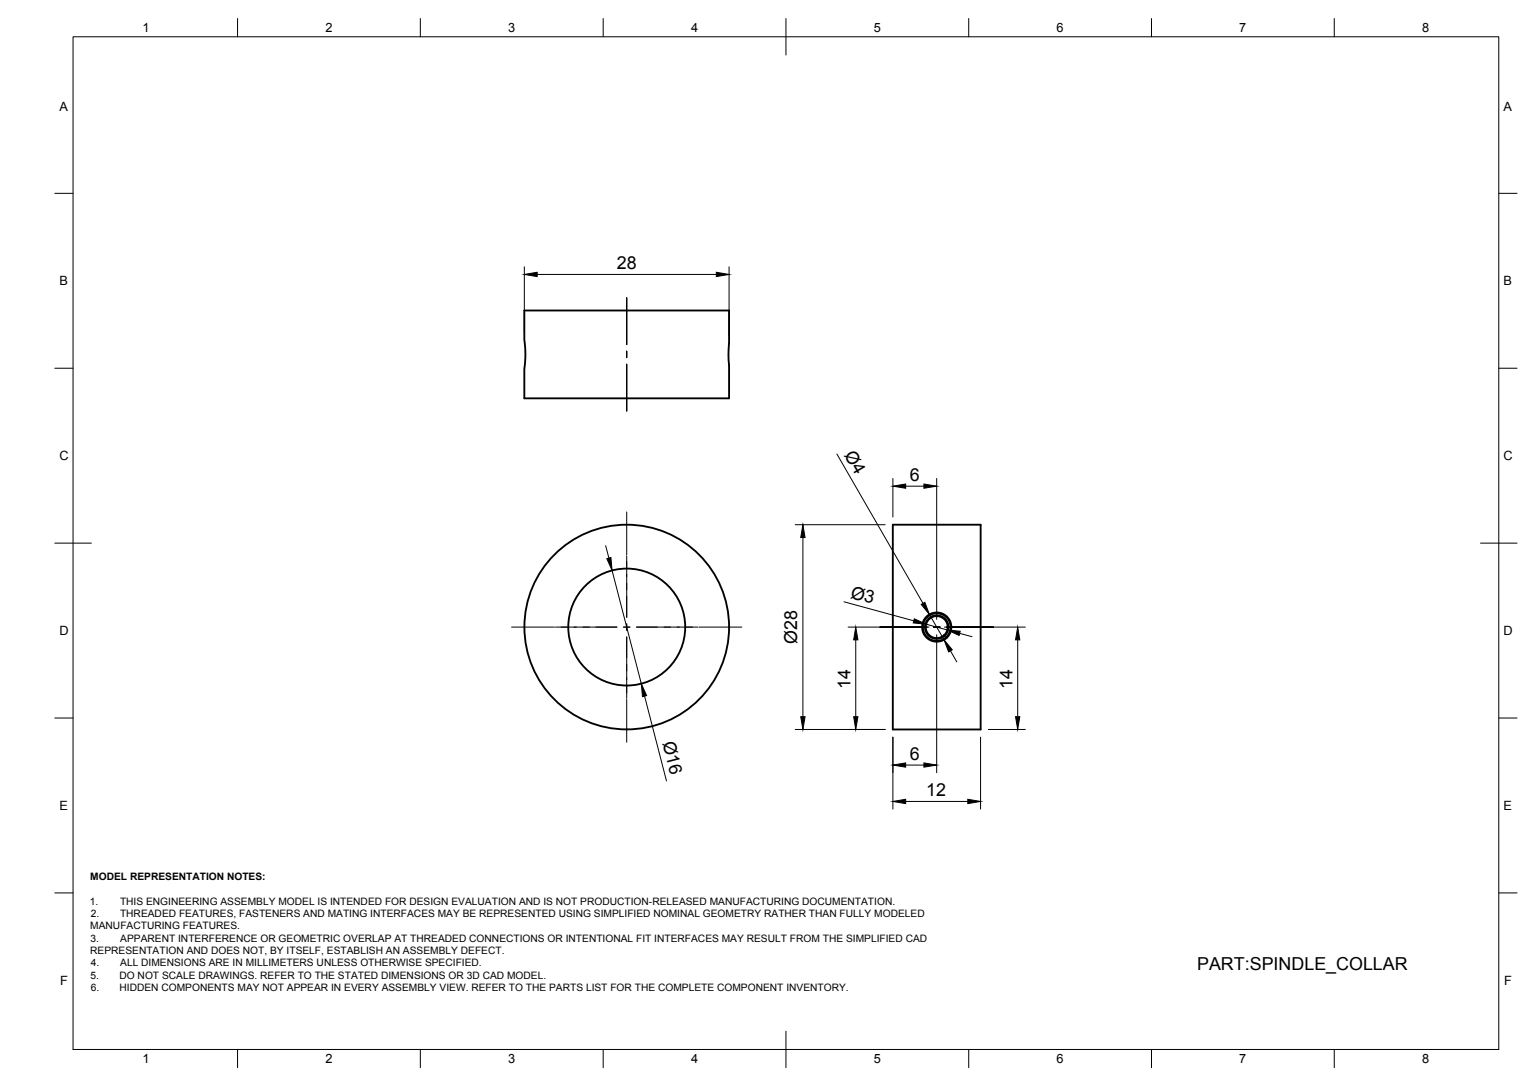
ISO-10303-21;
HEADER;
/* Generated by software containing ST-Developer
 * from STEP Tools, Inc. (www.steptools.com) 
 */

FILE_DESCRIPTION(
/* description */ (''),
/* implementation_level */ '2;1');

FILE_NAME(
/* name */ 'SPINDLE_COLLAR.step',
/* time_stamp */ '2026-10-04T02:10:06-07:00',
/* author */ (''),
/* organization */ (''),
/* preprocessor_version */ 'ST-DEVELOPER v20.2',
/* originating_system */ 'Autodesk Translation Framework v15.15.0.0',
/* authorisation */ '');

FILE_SCHEMA (('AUTOMOTIVE_DESIGN { 1 0 10303 214 3 1 1 }'));
ENDSEC;

DATA;
#10=MECHANICAL_DESIGN_GEOMETRIC_PRESENTATION_REPRESENTATION('',(#144),#9668);
#122=SHAPE_REPRESENTATION_RELATIONSHIP('SRR','None',#9715,#133);
#133=ADVANCED_BREP_SHAPE_REPRESENTATION('',(#155),#9660);
#144=STYLED_ITEM('',(#9775),#155);
#155=MANIFOLD_SOLID_BREP('Body1',#3884);
#170=CONICAL_SURFACE('',#4232,2.,0.0178552451395525);
#171=CONICAL_SURFACE('',#4233,2.,0.0178552451395525);
#237=FACE_BOUND('',#1171,.T.);
#238=FACE_BOUND('',#1173,.T.);
#239=FACE_BOUND('',#1175,.T.);
#240=FACE_BOUND('',#1177,.T.);
#311=PLANE('',#4224);
#312=PLANE('',#4227);
#466=LINE('',#6585,#657);
#467=LINE('',#6613,#658);
#468=LINE('',#6674,#659);
#469=LINE('',#6702,#660);
#470=LINE('',#6762,#661);
#471=LINE('',#6764,#662);
#657=VECTOR('',#4998,14.);
#658=VECTOR('',#4999,14.);
#659=VECTOR('',#5002,8.);
#660=VECTOR('',#5003,8.);
#661=VECTOR('',#5006,2.);
#662=VECTOR('',#5009,2.);
#790=CYLINDRICAL_SURFACE('',#4230,14.);
#791=CYLINDRICAL_SURFACE('',#4231,8.);
#905=FACE_OUTER_BOUND('',#1170,.T.);
#906=FACE_OUTER_BOUND('',#1172,.T.);
#907=FACE_OUTER_BOUND('',#1174,.T.);
#908=FACE_OUTER_BOUND('',#1176,.T.);
#909=FACE_OUTER_BOUND('',#1178,.T.);
#910=FACE_OUTER_BOUND('',#1179,.T.);
#1170=EDGE_LOOP('',(#3003));
#1171=EDGE_LOOP('',(#3004));
#1172=EDGE_LOOP('',(#3005));
#1173=EDGE_LOOP('',(#3006));
#1174=EDGE_LOOP('',(#3007,#3008,#3009,#3010,#3011,#3012,#3013,#3014,#3015,
#3016));
#1175=EDGE_LOOP('',(#3017,#3018));
#1176=EDGE_LOOP('',(#3019,#3020,#3021,#3022,#3023,#3024,#3025,#3026,#3027,
#3028));
#1177=EDGE_LOOP('',(#3029,#3030));
#1178=EDGE_LOOP('',(#3031,#3032,#3033,#3034,#3035,#3036,#3037,#3038,#3039,
#3040));
#1179=EDGE_LOOP('',(#3041,#3042,#3043,#3044,#3045,#3046));
#1347=B_SPLINE_CURVE_WITH_KNOTS('',3,(#6587,#6588,#6589,#6590,#6591,#6592,
#6593,#6594),.UNSPECIFIED.,.F.,.F.,(4,2,2,4),(0.904796449630696,0.980250998994914,
1.05570554835913,1.06208648908207),.UNSPECIFIED.);
#1348=B_SPLINE_CURVE_WITH_KNOTS('',3,(#6596,#6597,#6598,#6599,#6600,#6601),
 .UNSPECIFIED.,.F.,.F.,(4,2,4),(-0.144308777092194,-0.0753448589075656,
0.),.UNSPECIFIED.);
#1349=B_SPLINE_CURVE_WITH_KNOTS('',3,(#6603,#6604,#6605,#6606,#6607,#6608,
#6609,#6610,#6611,#6612),.UNSPECIFIED.,.F.,.F.,(4,2,2,2,4),(0.,0.0753448589075656,
0.150689717815131,0.226144267179348,0.301598816543565),.UNSPECIFIED.);
#1350=B_SPLINE_CURVE_WITH_KNOTS('',3,(#6614,#6615,#6616,#6617,#6618,#6619,
#6620,#6621,#6622,#6623,#6624,#6625,#6626,#6627,#6628,#6629,#6630,#6631),
 .UNSPECIFIED.,.F.,.F.,(4,2,2,2,2,2,2,2,4),(0.301598816543565,0.377053365907783,
0.452507915272,0.527852774179565,0.603197633087131,0.678542491994697,0.753887350902262,
0.829341900266479,0.904796449630696),.UNSPECIFIED.);
#1351=B_SPLINE_CURVE_WITH_KNOTS('',3,(#6634,#6635,#6636,#6637,#6638,#6639,
#6640,#6641,#6642,#6643,#6644,#6645,#6646,#6647,#6648,#6649,#6650,#6651,
#6652,#6653,#6654,#6655,#6656,#6657,#6658,#6659,#6660,#6661,#6662,#6663,
#6664,#6665),.UNSPECIFIED.,.F.,.F.,(4,2,2,2,2,2,2,2,2,2,2,2,2,2,2,4),(-0.795209907356727,
-0.792063991439152,-0.735493455630304,-0.678922919821455,-0.622352384012607,
-0.565781848203759,-0.509198564042365,-0.45261527988097,-0.396031995719576,
-0.339448711558182,-0.282878175749333,-0.226307639940485,-0.169737104131637,
-0.113166568322789,-0.0565832841613944,0.),.UNSPECIFIED.);
#1352=B_SPLINE_CURVE_WITH_KNOTS('',3,(#6666,#6667,#6668,#6669,#6670,#6671),
 .UNSPECIFIED.,.F.,.F.,(4,2,4),(0.,0.0565832841613945,0.110020652405213),
 .UNSPECIFIED.);
#1353=B_SPLINE_CURVE_WITH_KNOTS('',3,(#6676,#6677,#6678,#6679,#6680,#6681,
#6682,#6683,#6684,#6685),.UNSPECIFIED.,.F.,.F.,(4,2,2,2,4),(0.,0.0714283614509827,
0.142856722901965,0.214461611703495,0.286066500505024),.UNSPECIFIED.);
#1354=B_SPLINE_CURVE_WITH_KNOTS('',3,(#6687,#6688,#6689,#6690,#6691,#6692),
 .UNSPECIFIED.,.F.,.F.,(4,2,4),(-0.137591291556128,-0.0714283614509829,
0.),.UNSPECIFIED.);
#1355=B_SPLINE_CURVE_WITH_KNOTS('',3,(#6694,#6695,#6696,#6697,#6698,#6699,
#6700,#6701),.UNSPECIFIED.,.F.,.F.,(4,2,2,4),(0.858199501515072,0.929804390316601,
1.00140927911813,1.00667471046397),.UNSPECIFIED.);
#1356=B_SPLINE_CURVE_WITH_KNOTS('',3,(#6703,#6704,#6705,#6706,#6707,#6708,
#6709,#6710,#6711,#6712,#6713,#6714,#6715,#6716,#6717,#6718,#6719,#6720),
 .UNSPECIFIED.,.F.,.F.,(4,2,2,2,2,2,2,2,4),(0.286066500505024,0.357671389306553,
0.429276278108082,0.500704639559065,0.572133001010048,0.64356136246103,
0.714989723912013,0.786594612713542,0.858199501515072),.UNSPECIFIED.);
#1357=B_SPLINE_CURVE_WITH_KNOTS('',3,(#6723,#6724,#6725,#6726,#6727,#6728,
#6729,#6730,#6731,#6732,#6733,#6734,#6735,#6736,#6737,#6738,#6739,#6740,
#6741,#6742,#6743,#6744,#6745,#6746,#6747,#6748,#6749,#6750,#6751,#6752,
#6753,#6754),.UNSPECIFIED.,.F.,.F.,(4,2,2,2,2,2,2,2,2,2,2,2,2,2,2,4),(-0.856704581886595,
-0.85079361436338,-0.790035269749255,-0.72927692513513,-0.668518580521006,
-0.607760235906881,-0.546972426331817,-0.486184616756754,-0.42539680718169,
-0.364608997606626,-0.303850652992501,-0.243092308378377,-0.182333963764252,
-0.121575619150127,-0.0607878095750637,0.),.UNSPECIFIED.);
#1358=B_SPLINE_CURVE_WITH_KNOTS('',3,(#6755,#6756,#6757,#6758,#6759,#6760),
 .UNSPECIFIED.,.F.,.F.,(4,2,4),(0.,0.0607878095750638,0.115664651626913),
 .UNSPECIFIED.);
#1537=CIRCLE('',#4225,14.);
#1538=CIRCLE('',#4226,8.);
#1539=CIRCLE('',#4228,14.);
#1540=CIRCLE('',#4229,8.);
#1791=VERTEX_POINT('',#6574);
#1792=VERTEX_POINT('',#6576);
#1793=VERTEX_POINT('',#6579);
#1794=VERTEX_POINT('',#6581);
#1795=VERTEX_POINT('',#6584);
#1796=VERTEX_POINT('',#6586);
#1797=VERTEX_POINT('',#6595);
#1798=VERTEX_POINT('',#6602);
#1799=VERTEX_POINT('',#6632);
#1800=VERTEX_POINT('',#6633);
#1801=VERTEX_POINT('',#6673);
#1802=VERTEX_POINT('',#6675);
#1803=VERTEX_POINT('',#6686);
#1804=VERTEX_POINT('',#6693);
#1805=VERTEX_POINT('',#6721);
#1806=VERTEX_POINT('',#6722);
#2225=EDGE_CURVE('',#1791,#1791,#1537,.T.);
#2226=EDGE_CURVE('',#1792,#1792,#1538,.T.);
#2227=EDGE_CURVE('',#1793,#1793,#1539,.T.);
#2228=EDGE_CURVE('',#1794,#1794,#1540,.T.);
#2229=EDGE_CURVE('',#1793,#1795,#466,.T.);
#2230=EDGE_CURVE('',#1795,#1796,#1347,.T.);
#2231=EDGE_CURVE('',#1796,#1797,#1348,.T.);
#2232=EDGE_CURVE('',#1797,#1798,#1349,.T.);
#2233=EDGE_CURVE('',#1798,#1791,#467,.T.);
#2234=EDGE_CURVE('',#1798,#1795,#1350,.T.);
#2235=EDGE_CURVE('',#1799,#1800,#1351,.T.);
#2236=EDGE_CURVE('',#1800,#1799,#1352,.T.);
#2237=EDGE_CURVE('',#1792,#1801,#468,.T.);
#2238=EDGE_CURVE('',#1802,#1801,#1353,.T.);
#2239=EDGE_CURVE('',#1803,#1802,#1354,.T.);
#2240=EDGE_CURVE('',#1804,#1803,#1355,.T.);
#2241=EDGE_CURVE('',#1804,#1794,#469,.T.);
#2242=EDGE_CURVE('',#1801,#1804,#1356,.T.);
#2243=EDGE_CURVE('',#1805,#1806,#1357,.T.);
#2244=EDGE_CURVE('',#1806,#1805,#1358,.T.);
#2245=EDGE_CURVE('',#1802,#1797,#470,.T.);
#2246=EDGE_CURVE('',#1800,#1806,#471,.T.);
#3003=ORIENTED_EDGE('',*,*,#2225,.T.);
#3004=ORIENTED_EDGE('',*,*,#2226,.F.);
#3005=ORIENTED_EDGE('',*,*,#2227,.F.);
#3006=ORIENTED_EDGE('',*,*,#2228,.T.);
#3007=ORIENTED_EDGE('',*,*,#2227,.T.);
#3008=ORIENTED_EDGE('',*,*,#2229,.T.);
#3009=ORIENTED_EDGE('',*,*,#2230,.T.);
#3010=ORIENTED_EDGE('',*,*,#2231,.T.);
#3011=ORIENTED_EDGE('',*,*,#2232,.T.);
#3012=ORIENTED_EDGE('',*,*,#2233,.T.);
#3013=ORIENTED_EDGE('',*,*,#2225,.F.);
#3014=ORIENTED_EDGE('',*,*,#2233,.F.);
#3015=ORIENTED_EDGE('',*,*,#2234,.T.);
#3016=ORIENTED_EDGE('',*,*,#2229,.F.);
#3017=ORIENTED_EDGE('',*,*,#2235,.T.);
#3018=ORIENTED_EDGE('',*,*,#2236,.T.);
#3019=ORIENTED_EDGE('',*,*,#2226,.T.);
#3020=ORIENTED_EDGE('',*,*,#2237,.T.);
#3021=ORIENTED_EDGE('',*,*,#2238,.F.);
#3022=ORIENTED_EDGE('',*,*,#2239,.F.);
#3023=ORIENTED_EDGE('',*,*,#2240,.F.);
#3024=ORIENTED_EDGE('',*,*,#2241,.T.);
#3025=ORIENTED_EDGE('',*,*,#2228,.F.);
#3026=ORIENTED_EDGE('',*,*,#2241,.F.);
#3027=ORIENTED_EDGE('',*,*,#2242,.F.);
#3028=ORIENTED_EDGE('',*,*,#2237,.F.);
#3029=ORIENTED_EDGE('',*,*,#2243,.F.);
#3030=ORIENTED_EDGE('',*,*,#2244,.F.);
#3031=ORIENTED_EDGE('',*,*,#2239,.T.);
#3032=ORIENTED_EDGE('',*,*,#2245,.T.);
#3033=ORIENTED_EDGE('',*,*,#2231,.F.);
#3034=ORIENTED_EDGE('',*,*,#2230,.F.);
#3035=ORIENTED_EDGE('',*,*,#2234,.F.);
#3036=ORIENTED_EDGE('',*,*,#2232,.F.);
#3037=ORIENTED_EDGE('',*,*,#2245,.F.);
#3038=ORIENTED_EDGE('',*,*,#2238,.T.);
#3039=ORIENTED_EDGE('',*,*,#2242,.T.);
#3040=ORIENTED_EDGE('',*,*,#2240,.T.);
#3041=ORIENTED_EDGE('',*,*,#2235,.F.);
#3042=ORIENTED_EDGE('',*,*,#2236,.F.);
#3043=ORIENTED_EDGE('',*,*,#2246,.T.);
#3044=ORIENTED_EDGE('',*,*,#2244,.T.);
#3045=ORIENTED_EDGE('',*,*,#2243,.T.);
#3046=ORIENTED_EDGE('',*,*,#2246,.F.);
#3753=ADVANCED_FACE('',(#905,#237),#311,.T.);
#3754=ADVANCED_FACE('',(#906,#238),#312,.F.);
#3755=ADVANCED_FACE('',(#907,#239),#790,.T.);
#3756=ADVANCED_FACE('',(#908,#240),#791,.F.);
#3757=ADVANCED_FACE('',(#909),#170,.F.);
#3758=ADVANCED_FACE('',(#910),#171,.F.);
#3884=CLOSED_SHELL('',(#3753,#3754,#3755,#3756,#3757,#3758));
#4223=AXIS2_PLACEMENT_3D('',#6572,#4982,#4983);
#4224=AXIS2_PLACEMENT_3D('',#6573,#4984,#4985);
#4225=AXIS2_PLACEMENT_3D('',#6575,#4986,#4987);
#4226=AXIS2_PLACEMENT_3D('',#6577,#4988,#4989);
#4227=AXIS2_PLACEMENT_3D('',#6578,#4990,#4991);
#4228=AXIS2_PLACEMENT_3D('',#6580,#4992,#4993);
#4229=AXIS2_PLACEMENT_3D('',#6582,#4994,#4995);
#4230=AXIS2_PLACEMENT_3D('',#6583,#4996,#4997);
#4231=AXIS2_PLACEMENT_3D('',#6672,#5000,#5001);
#4232=AXIS2_PLACEMENT_3D('',#6761,#5004,#5005);
#4233=AXIS2_PLACEMENT_3D('',#6763,#5007,#5008);
#4982=DIRECTION('axis',(0.,0.,1.));
#4983=DIRECTION('refdir',(1.,0.,0.));
#4984=DIRECTION('center_axis',(0.,1.,0.));
#4985=DIRECTION('ref_axis',(0.,0.,1.));
#4986=DIRECTION('center_axis',(0.,1.,0.));
#4987=DIRECTION('ref_axis',(0.,0.,1.));
#4988=DIRECTION('center_axis',(0.,1.,0.));
#4989=DIRECTION('ref_axis',(0.,0.,1.));
#4990=DIRECTION('center_axis',(0.,1.,0.));
#4991=DIRECTION('ref_axis',(0.,0.,1.));
#4992=DIRECTION('center_axis',(0.,1.,0.));
#4993=DIRECTION('ref_axis',(0.,0.,1.));
#4994=DIRECTION('center_axis',(0.,1.,0.));
#4995=DIRECTION('ref_axis',(0.,0.,1.));
#4996=DIRECTION('center_axis',(0.,-1.,0.));
#4997=DIRECTION('ref_axis',(0.,0.,-1.));
#4998=DIRECTION('',(0.,1.,0.));
#4999=DIRECTION('',(0.,1.,0.));
#5000=DIRECTION('center_axis',(0.,-1.,0.));
#5001=DIRECTION('ref_axis',(0.,0.,-1.));
#5002=DIRECTION('',(0.,-1.,0.));
#5003=DIRECTION('',(0.,-1.,0.));
#5004=DIRECTION('center_axis',(0.,0.,1.));
#5005=DIRECTION('ref_axis',(1.,0.,0.));
#5006=DIRECTION('',(-0.017854296416883,-2.18652069579638E-18,0.999840599345445));
#5007=DIRECTION('center_axis',(0.,0.,1.));
#5008=DIRECTION('ref_axis',(1.,0.,0.));
#5009=DIRECTION('',(-0.017854296416883,-2.18652069579638E-18,0.999840599345445));
#6572=CARTESIAN_POINT('',(0.,0.,0.));
#6573=CARTESIAN_POINT('Origin',(0.,12.,0.));
#6574=CARTESIAN_POINT('',(0.,12.,14.));
#6575=CARTESIAN_POINT('Origin',(0.,12.,0.));
#6576=CARTESIAN_POINT('',(0.,12.,8.));
#6577=CARTESIAN_POINT('Origin',(0.,12.,0.));
#6578=CARTESIAN_POINT('Origin',(0.,0.,0.));
#6579=CARTESIAN_POINT('',(0.,0.,14.));
#6580=CARTESIAN_POINT('Origin',(0.,0.,0.));
#6581=CARTESIAN_POINT('',(0.,0.,8.));
#6582=CARTESIAN_POINT('Origin',(0.,0.,0.));
#6583=CARTESIAN_POINT('Origin',(0.,12.,0.));
#6584=CARTESIAN_POINT('',(-8.22558289883611E-16,4.,14.));
#6585=CARTESIAN_POINT('',(-1.71450551880629E-15,12.,14.));
#6586=CARTESIAN_POINT('',(-1.45802973181661,4.63299112089927,13.9238697674583));
#6587=CARTESIAN_POINT('Ctrl Pts',(6.93889390390723E-17,4.,14.));
#6588=CARTESIAN_POINT('Ctrl Pts',(-0.25151516454739,4.,14.));
#6589=CARTESIAN_POINT('Ctrl Pts',(-0.519513937917108,4.050469286675,13.9925306456456));
#6590=CARTESIAN_POINT('Ctrl Pts',(-1.01196367232324,4.25513100778376,13.9655554177696));
#6591=CARTESIAN_POINT('Ctrl Pts',(-1.23644395127912,4.40930284567681,13.9464298471224));
#6592=CARTESIAN_POINT('Ctrl Pts',(-1.42855606179944,4.60197987136062,13.9269326944353));
#6593=CARTESIAN_POINT('Ctrl Pts',(-1.44338181871977,4.61732784601981,13.9254036149562));
#6594=CARTESIAN_POINT('Ctrl Pts',(-1.45802973181661,4.63299112089927,13.9238697674583));
#6595=CARTESIAN_POINT('',(-1.99744241740809,6.,13.8567753748532));
#6596=CARTESIAN_POINT('Ctrl Pts',(-1.45802973181661,4.63299112089927,13.9238697674583));
#6597=CARTESIAN_POINT('Ctrl Pts',(-1.61634141723231,4.80227663132682,13.9072922535857));
#6598=CARTESIAN_POINT('Ctrl Pts',(-1.75242809682337,5.00975783196893,13.8902060158894));
#6599=CARTESIAN_POINT('Ctrl Pts',(-1.94731439399108,5.48114930972434,13.8642887746891));
#6600=CARTESIAN_POINT('Ctrl Pts',(-1.99744241740809,5.74885047030811,13.8567753748532));
#6601=CARTESIAN_POINT('Ctrl Pts',(-1.99744241740809,6.,13.8567753748532));
#6602=CARTESIAN_POINT('',(-7.87863820364075E-16,8.,14.));
#6603=CARTESIAN_POINT('Ctrl Pts',(-1.99744241740809,6.,13.8567753748532));
#6604=CARTESIAN_POINT('Ctrl Pts',(-1.99744241740809,6.25114952969189,13.8567753748532));
#6605=CARTESIAN_POINT('Ctrl Pts',(-1.94731439399108,6.51885069027566,13.8642887746891));
#6606=CARTESIAN_POINT('Ctrl Pts',(-1.74381075604205,7.01108581411736,13.8913520056423));
#6607=CARTESIAN_POINT('Ctrl Pts',(-1.59045163862178,7.23564848986549,13.9105021697166));
#6608=CARTESIAN_POINT('Ctrl Pts',(-1.23644395127912,7.59069715432319,13.9464298471224));
#6609=CARTESIAN_POINT('Ctrl Pts',(-1.01196367232324,7.74486899221624,13.9655554177696));
#6610=CARTESIAN_POINT('Ctrl Pts',(-0.519513937917107,7.949530713325,13.9925306456456));
#6611=CARTESIAN_POINT('Ctrl Pts',(-0.25151516454739,8.,14.));
#6612=CARTESIAN_POINT('Ctrl Pts',(1.38777878078145E-16,8.,14.));
#6613=CARTESIAN_POINT('',(-1.71450551880629E-15,12.,14.));
#6614=CARTESIAN_POINT('Ctrl Pts',(2.08166817117217E-16,8.,14.));
#6615=CARTESIAN_POINT('Ctrl Pts',(0.251515164547391,8.,14.));
#6616=CARTESIAN_POINT('Ctrl Pts',(0.519513937917107,7.949530713325,13.9925306456456));
#6617=CARTESIAN_POINT('Ctrl Pts',(1.01196367232324,7.74486899221624,13.9655554177696));
#6618=CARTESIAN_POINT('Ctrl Pts',(1.23644395127912,7.59069715432319,13.9464298471224));
#6619=CARTESIAN_POINT('Ctrl Pts',(1.59045163862178,7.23564848986549,13.9105021697166));
#6620=CARTESIAN_POINT('Ctrl Pts',(1.74381075604205,7.01108581411736,13.8913520056423));
#6621=CARTESIAN_POINT('Ctrl Pts',(1.94731439399108,6.51885069027566,13.8642887746891));
#6622=CARTESIAN_POINT('Ctrl Pts',(1.99744241740809,6.25114952969188,13.8567753748532));
#6623=CARTESIAN_POINT('Ctrl Pts',(1.99744241740809,5.74885047030811,13.8567753748532));
#6624=CARTESIAN_POINT('Ctrl Pts',(1.94731439399108,5.48114930972434,13.8642887746891));
#6625=CARTESIAN_POINT('Ctrl Pts',(1.74381075604205,4.98891418588264,13.8913520056423));
#6626=CARTESIAN_POINT('Ctrl Pts',(1.59045163862178,4.76435151013451,13.9105021697166));
#6627=CARTESIAN_POINT('Ctrl Pts',(1.23644395127912,4.40930284567681,13.9464298471224));
#6628=CARTESIAN_POINT('Ctrl Pts',(1.01196367232324,4.25513100778376,13.9655554177696));
#6629=CARTESIAN_POINT('Ctrl Pts',(0.519513937917108,4.050469286675,13.9925306456456));
#6630=CARTESIAN_POINT('Ctrl Pts',(0.251515164547391,4.,14.));
#6631=CARTESIAN_POINT('Ctrl Pts',(2.08166817117217E-16,4.,14.));
#6632=CARTESIAN_POINT('',(-1.08344435620045,4.96154049110382,-13.9580137672599));
#6633=CARTESIAN_POINT('',(-1.50144186694001,6.,-13.9192554513594));
#6634=CARTESIAN_POINT('Ctrl Pts',(-1.08344435620045,4.96154049110382,-13.9580137672599));
#6635=CARTESIAN_POINT('Ctrl Pts',(-1.0761391389456,4.95393345386291,-13.9585808104322));
#6636=CARTESIAN_POINT('Ctrl Pts',(-1.06877893978868,4.94642971506651,-13.9591463493795));
#6637=CARTESIAN_POINT('Ctrl Pts',(-0.928120699239766,4.80598855727717,-13.969840718405));
#6638=CARTESIAN_POINT('Ctrl Pts',(-0.75939870112794,4.69065402980549,-13.980613498328));
#6639=CARTESIAN_POINT('Ctrl Pts',(-0.389628419705622,4.53765624525252,-13.9958004369066));
#6640=CARTESIAN_POINT('Ctrl Pts',(-0.18856845269616,4.5,-14.));
#6641=CARTESIAN_POINT('Ctrl Pts',(0.188568452696161,4.5,-14.));
#6642=CARTESIAN_POINT('Ctrl Pts',(0.389628419705623,4.53765624525252,-13.9958004369066));
#6643=CARTESIAN_POINT('Ctrl Pts',(0.75939870112794,4.69065402980549,-13.980613498328));
#6644=CARTESIAN_POINT('Ctrl Pts',(0.928120699239766,4.80598855727717,-13.969840718405));
#6645=CARTESIAN_POINT('Ctrl Pts',(1.19464720522372,5.07210372362547,-13.9495764750947));
#6646=CARTESIAN_POINT('Ctrl Pts',(1.31025681386282,5.24069144342751,-13.9387649526973));
#6647=CARTESIAN_POINT('Ctrl Pts',(1.4636586514978,5.61032763153242,-13.9234925472081));
#6648=CARTESIAN_POINT('Ctrl Pts',(1.50144186694001,5.81138905279535,-13.9192554513594));
#6649=CARTESIAN_POINT('Ctrl Pts',(1.50144186694001,6.18861094720465,-13.9192554513594));
#6650=CARTESIAN_POINT('Ctrl Pts',(1.4636586514978,6.38967236846757,-13.9234925472081));
#6651=CARTESIAN_POINT('Ctrl Pts',(1.31025681386282,6.75930855657249,-13.9387649526973));
#6652=CARTESIAN_POINT('Ctrl Pts',(1.19464720522372,6.92789627637453,-13.9495764750947));
#6653=CARTESIAN_POINT('Ctrl Pts',(0.928120699239766,7.19401144272283,-13.969840718405));
#6654=CARTESIAN_POINT('Ctrl Pts',(0.75939870112794,7.30934597019451,-13.980613498328));
#6655=CARTESIAN_POINT('Ctrl Pts',(0.389628419705623,7.46234375474748,-13.9958004369066));
#6656=CARTESIAN_POINT('Ctrl Pts',(0.188568452696161,7.5,-14.));
#6657=CARTESIAN_POINT('Ctrl Pts',(-0.188568452696161,7.5,-14.));
#6658=CARTESIAN_POINT('Ctrl Pts',(-0.389628419705623,7.46234375474748,-13.9958004369066));
#6659=CARTESIAN_POINT('Ctrl Pts',(-0.75939870112794,7.30934597019451,-13.980613498328));
#6660=CARTESIAN_POINT('Ctrl Pts',(-0.928120699239766,7.19401144272283,-13.969840718405));
#6661=CARTESIAN_POINT('Ctrl Pts',(-1.19464720522372,6.92789627637453,-13.9495764750947));
#6662=CARTESIAN_POINT('Ctrl Pts',(-1.31025681386282,6.75930855657249,-13.9387649526973));
#6663=CARTESIAN_POINT('Ctrl Pts',(-1.4636586514978,6.38967236846757,-13.9234925472081));
#6664=CARTESIAN_POINT('Ctrl Pts',(-1.50144186694001,6.18861094720465,-13.9192554513594));
#6665=CARTESIAN_POINT('Ctrl Pts',(-1.50144186694001,6.,-13.9192554513594));
#6666=CARTESIAN_POINT('Ctrl Pts',(-1.50144186694001,6.,-13.9192554513594));
#6667=CARTESIAN_POINT('Ctrl Pts',(-1.50144186694001,5.81138905279535,-13.9192554513594));
#6668=CARTESIAN_POINT('Ctrl Pts',(-1.4636586514978,5.61032763153242,-13.9234925472081));
#6669=CARTESIAN_POINT('Ctrl Pts',(-1.31452122949328,5.25096695487144,-13.9383403953016));
#6670=CARTESIAN_POINT('Ctrl Pts',(-1.20753272816477,5.09075565798599,-13.9483818204431));
#6671=CARTESIAN_POINT('Ctrl Pts',(-1.08344435620045,4.96154049110382,-13.9580137672599));
#6672=CARTESIAN_POINT('Origin',(0.,12.,0.));
#6673=CARTESIAN_POINT('',(-4.89858719658941E-16,7.89285714285714,8.));
#6674=CARTESIAN_POINT('',(-9.79717439317883E-16,12.,8.));
#6675=CARTESIAN_POINT('',(-1.8888183153337,6.,7.77382565868698));
#6676=CARTESIAN_POINT('Ctrl Pts',(-1.8888183153337,6.,7.77382565868698));
#6677=CARTESIAN_POINT('Ctrl Pts',(-1.8888183153337,6.23809453816994,7.77382565868698));
#6678=CARTESIAN_POINT('Ctrl Pts',(-1.84126818534383,6.49149873782234,7.78584860900432));
#6679=CARTESIAN_POINT('Ctrl Pts',(-1.64896551578976,6.95689762810345,7.8288325824729));
#6680=CARTESIAN_POINT('Ctrl Pts',(-1.50425576119276,7.16897165737161,7.85912333726051));
#6681=CARTESIAN_POINT('Ctrl Pts',(-1.17034427142268,7.50455135351629,7.91574638772443));
#6682=CARTESIAN_POINT('Ctrl Pts',(-0.958382508360478,7.65058083501241,7.94582869803651));
#6683=CARTESIAN_POINT('Ctrl Pts',(-0.492588734304788,7.84475933338953,7.98824430458773));
#6684=CARTESIAN_POINT('Ctrl Pts',(-0.238682962671764,7.89285714285714,8.));
#6685=CARTESIAN_POINT('Ctrl Pts',(6.93889390390723E-17,7.89285714285714,
8.));
#6686=CARTESIAN_POINT('',(-1.37403979594041,4.70119646738038,7.88111760089723));
#6687=CARTESIAN_POINT('Ctrl Pts',(-1.37403979594041,4.70119646738038,7.88111760089723));
#6688=CARTESIAN_POINT('Ctrl Pts',(-1.52556322669951,4.86218398763909,7.85470012631764));
#6689=CARTESIAN_POINT('Ctrl Pts',(-1.65605343215512,5.06025610365957,7.82724827368664));
#6690=CARTESIAN_POINT('Ctrl Pts',(-1.84126818534383,5.50850126217766,7.78584860900432));
#6691=CARTESIAN_POINT('Ctrl Pts',(-1.8888183153337,5.76190546183006,7.77382565868698));
#6692=CARTESIAN_POINT('Ctrl Pts',(-1.8888183153337,6.,7.77382565868698));
#6693=CARTESIAN_POINT('',(-7.32720006295694E-16,4.10714285714286,8.));
#6694=CARTESIAN_POINT('Ctrl Pts',(0.,4.10714285714286,8.));
#6695=CARTESIAN_POINT('Ctrl Pts',(-0.238682962671764,4.10714285714286,8.));
#6696=CARTESIAN_POINT('Ctrl Pts',(-0.492588734304787,4.15524066661047,7.98824430458773));
#6697=CARTESIAN_POINT('Ctrl Pts',(-0.958382508360477,4.34941916498759,7.94582869803651));
#6698=CARTESIAN_POINT('Ctrl Pts',(-1.17034427142268,4.49544864648371,7.91574638772443));
#6699=CARTESIAN_POINT('Ctrl Pts',(-1.34979823107329,4.67579914982511,7.88531547736479));
#6700=CARTESIAN_POINT('Ctrl Pts',(-1.3619811367988,4.68838462948094,7.88321997753786));
#6701=CARTESIAN_POINT('Ctrl Pts',(-1.37403979594041,4.70119646738038,7.88111760089723));
#6702=CARTESIAN_POINT('',(-9.79717439317883E-16,12.,8.));
#6703=CARTESIAN_POINT('Ctrl Pts',(6.93889390390723E-17,7.89285714285714,
8.));
#6704=CARTESIAN_POINT('Ctrl Pts',(0.238682962671764,7.89285714285714,8.));
#6705=CARTESIAN_POINT('Ctrl Pts',(0.492588734304788,7.84475933338953,7.98824430458773));
#6706=CARTESIAN_POINT('Ctrl Pts',(0.958382508360478,7.65058083501241,7.94582869803651));
#6707=CARTESIAN_POINT('Ctrl Pts',(1.17034427142268,7.50455135351629,7.91574638772443));
#6708=CARTESIAN_POINT('Ctrl Pts',(1.50425576119275,7.16897165737161,7.85912333726051));
#6709=CARTESIAN_POINT('Ctrl Pts',(1.64896551578976,6.95689762810345,7.8288325824729));
#6710=CARTESIAN_POINT('Ctrl Pts',(1.84126818534383,6.49149873782234,7.78584860900432));
#6711=CARTESIAN_POINT('Ctrl Pts',(1.8888183153337,6.23809453816994,7.77382565868698));
#6712=CARTESIAN_POINT('Ctrl Pts',(1.8888183153337,5.76190546183006,7.77382565868698));
#6713=CARTESIAN_POINT('Ctrl Pts',(1.84126818534383,5.50850126217766,7.78584860900432));
#6714=CARTESIAN_POINT('Ctrl Pts',(1.64896551578976,5.04310237189655,7.8288325824729));
#6715=CARTESIAN_POINT('Ctrl Pts',(1.50425576119275,4.83102834262839,7.85912333726051));
#6716=CARTESIAN_POINT('Ctrl Pts',(1.17034427142268,4.49544864648371,7.91574638772443));
#6717=CARTESIAN_POINT('Ctrl Pts',(0.958382508360478,4.34941916498759,7.94582869803651));
#6718=CARTESIAN_POINT('Ctrl Pts',(0.492588734304788,4.15524066661047,7.98824430458773));
#6719=CARTESIAN_POINT('Ctrl Pts',(0.238682962671764,4.10714285714286,8.));
#6720=CARTESIAN_POINT('Ctrl Pts',(-2.77555756156289E-16,4.10714285714286,
8.));
#6721=CARTESIAN_POINT('',(-1.17898168752143,4.90550167217474,-7.91264824066438));
#6722=CARTESIAN_POINT('',(-1.61006596901441,6.,-7.83630573519319));
#6723=CARTESIAN_POINT('Ctrl Pts',(-1.17898168752143,4.90550167217474,-7.91264824066438));
#6724=CARTESIAN_POINT('Ctrl Pts',(-1.16545353798237,4.89098220165951,-7.91466392998703));
#6725=CARTESIAN_POINT('Ctrl Pts',(-1.15173426773385,4.87679671704893,-7.91667258611177));
#6726=CARTESIAN_POINT('Ctrl Pts',(-0.995172181265423,4.72069148871753,-7.93916938835585));
#6727=CARTESIAN_POINT('Ctrl Pts',(-0.814524503839801,4.5972583768551,-7.96090747080436));
#6728=CARTESIAN_POINT('Ctrl Pts',(-0.418224335279089,4.43332696536825,-7.99153216392396));
#6729=CARTESIAN_POINT('Ctrl Pts',(-0.202527815380415,4.39285714285714,-8.));
#6730=CARTESIAN_POINT('Ctrl Pts',(0.202527815380416,4.39285714285714,-8.));
#6731=CARTESIAN_POINT('Ctrl Pts',(0.418224335279089,4.43332696536825,-7.99153216392396));
#6732=CARTESIAN_POINT('Ctrl Pts',(0.814524503839801,4.5972583768551,-7.96090747080436));
#6733=CARTESIAN_POINT('Ctrl Pts',(0.995172181265423,4.72069148871753,-7.93916938835585));
#6734=CARTESIAN_POINT('Ctrl Pts',(1.28060364728793,5.00529004754802,-7.89815501897568));
#6735=CARTESIAN_POINT('Ctrl Pts',(1.40458789962237,5.18566238393601,-7.876176798428));
#6736=CARTESIAN_POINT('Ctrl Pts',(1.5693348410951,5.58167896973006,-7.84501220025286));
#6737=CARTESIAN_POINT('Ctrl Pts',(1.61006596901441,5.79737396808312,-7.83630573519319));
#6738=CARTESIAN_POINT('Ctrl Pts',(1.61006596901441,6.20262603191688,-7.83630573519319));
#6739=CARTESIAN_POINT('Ctrl Pts',(1.5693348410951,6.41832103026994,-7.84501220025286));
#6740=CARTESIAN_POINT('Ctrl Pts',(1.40458789962237,6.81433761606399,-7.876176798428));
#6741=CARTESIAN_POINT('Ctrl Pts',(1.28060364728793,6.99470995245198,-7.89815501897568));
#6742=CARTESIAN_POINT('Ctrl Pts',(0.995172181265423,7.27930851128247,-7.93916938835585));
#6743=CARTESIAN_POINT('Ctrl Pts',(0.814524503839801,7.4027416231449,-7.96090747080436));
#6744=CARTESIAN_POINT('Ctrl Pts',(0.418224335279089,7.56667303463175,-7.99153216392396));
#6745=CARTESIAN_POINT('Ctrl Pts',(0.202527815380415,7.60714285714286,-8.));
#6746=CARTESIAN_POINT('Ctrl Pts',(-0.202527815380416,7.60714285714286,-8.));
#6747=CARTESIAN_POINT('Ctrl Pts',(-0.41822433527909,7.56667303463175,-7.99153216392396));
#6748=CARTESIAN_POINT('Ctrl Pts',(-0.814524503839802,7.4027416231449,-7.96090747080436));
#6749=CARTESIAN_POINT('Ctrl Pts',(-0.995172181265423,7.27930851128247,-7.93916938835585));
#6750=CARTESIAN_POINT('Ctrl Pts',(-1.28060364728793,6.99470995245198,-7.89815501897568));
#6751=CARTESIAN_POINT('Ctrl Pts',(-1.40458789962237,6.81433761606399,-7.876176798428));
#6752=CARTESIAN_POINT('Ctrl Pts',(-1.5693348410951,6.41832103026994,-7.84501220025286));
#6753=CARTESIAN_POINT('Ctrl Pts',(-1.61006596901441,6.20262603191688,-7.83630573519319));
#6754=CARTESIAN_POINT('Ctrl Pts',(-1.61006596901441,6.,-7.83630573519319));
#6755=CARTESIAN_POINT('Ctrl Pts',(-1.61006596901441,6.,-7.83630573519319));
#6756=CARTESIAN_POINT('Ctrl Pts',(-1.61006596901441,5.79737396808312,-7.83630573519319));
#6757=CARTESIAN_POINT('Ctrl Pts',(-1.5693348410951,5.58167896973006,-7.84501220025286));
#6758=CARTESIAN_POINT('Ctrl Pts',(-1.41259784295971,5.2049165830398,-7.87466158568243));
#6759=CARTESIAN_POINT('Ctrl Pts',(-1.30457569943121,5.04029901068342,-7.89393477892562));
#6760=CARTESIAN_POINT('Ctrl Pts',(-1.17898168752143,4.90550167217474,-7.91264824066438));
#6761=CARTESIAN_POINT('Origin',(0.,6.,14.));
#6762=CARTESIAN_POINT('',(-2.,6.,14.));
#6763=CARTESIAN_POINT('Origin',(0.,6.,14.));
#6764=CARTESIAN_POINT('',(-2.,6.,14.));
#9647=UNCERTAINTY_MEASURE_WITH_UNIT(LENGTH_MEASURE(0.01),#9669,
'DISTANCE_ACCURACY_VALUE',
'Maximum model space distance between geometric entities at asserted c
onnectivities');
#9655=UNCERTAINTY_MEASURE_WITH_UNIT(LENGTH_MEASURE(0.01),#9669,
'DISTANCE_ACCURACY_VALUE',
'Maximum model space distance between geometric entities at asserted c
onnectivities');
#9660=(
GEOMETRIC_REPRESENTATION_CONTEXT(3)
GLOBAL_UNCERTAINTY_ASSIGNED_CONTEXT((#9647))
GLOBAL_UNIT_ASSIGNED_CONTEXT((#9669,#9671,#9672))
REPRESENTATION_CONTEXT('','3D')
);
#9668=(
GEOMETRIC_REPRESENTATION_CONTEXT(3)
GLOBAL_UNCERTAINTY_ASSIGNED_CONTEXT((#9655))
GLOBAL_UNIT_ASSIGNED_CONTEXT((#9669,#9671,#9672))
REPRESENTATION_CONTEXT('','3D')
);
#9669=(
LENGTH_UNIT()
NAMED_UNIT(*)
SI_UNIT(.MILLI.,.METRE.)
);
#9671=(
NAMED_UNIT(*)
PLANE_ANGLE_UNIT()
SI_UNIT($,.RADIAN.)
);
#9672=(
NAMED_UNIT(*)
SI_UNIT($,.STERADIAN.)
SOLID_ANGLE_UNIT()
);
#9677=SHAPE_DEFINITION_REPRESENTATION(#9689,#9715);
#9689=PRODUCT_DEFINITION_SHAPE('',$,#9728);
#9715=SHAPE_REPRESENTATION('',(#4223),#9660);
#9723=PRODUCT_DEFINITION_CONTEXT('part definition',#9761,'design');
#9728=PRODUCT_DEFINITION('2026-10-04-08-13-48-883','SPINDLE_COLLAR',#9740,
#9723);
#9740=PRODUCT_DEFINITION_FORMATION('',$,#9767);
#9761=APPLICATION_CONTEXT(
'Core Data for Automotive Mechanical Design Process');
#9762=PRODUCT_CONTEXT('part definition',#9761,'mechanical');
#9767=PRODUCT('2026-10-04-08-13-48-883','SPINDLE_COLLAR','PART',(#9762));
#9775=PRESENTATION_STYLE_ASSIGNMENT((#9776));
#9776=SURFACE_STYLE_USAGE(.BOTH.,#9777);
#9777=SURFACE_SIDE_STYLE('',(#9778));
#9778=SURFACE_STYLE_FILL_AREA(#9779);
#9779=FILL_AREA_STYLE('Steel - Satin',(#9780));
#9780=FILL_AREA_STYLE_COLOUR('Steel - Satin',#9781);
#9781=COLOUR_RGB('Steel - Satin', 0.09019608, 0.27058824, 0.51372549);
ENDSEC;
END-ISO-10303-21;
